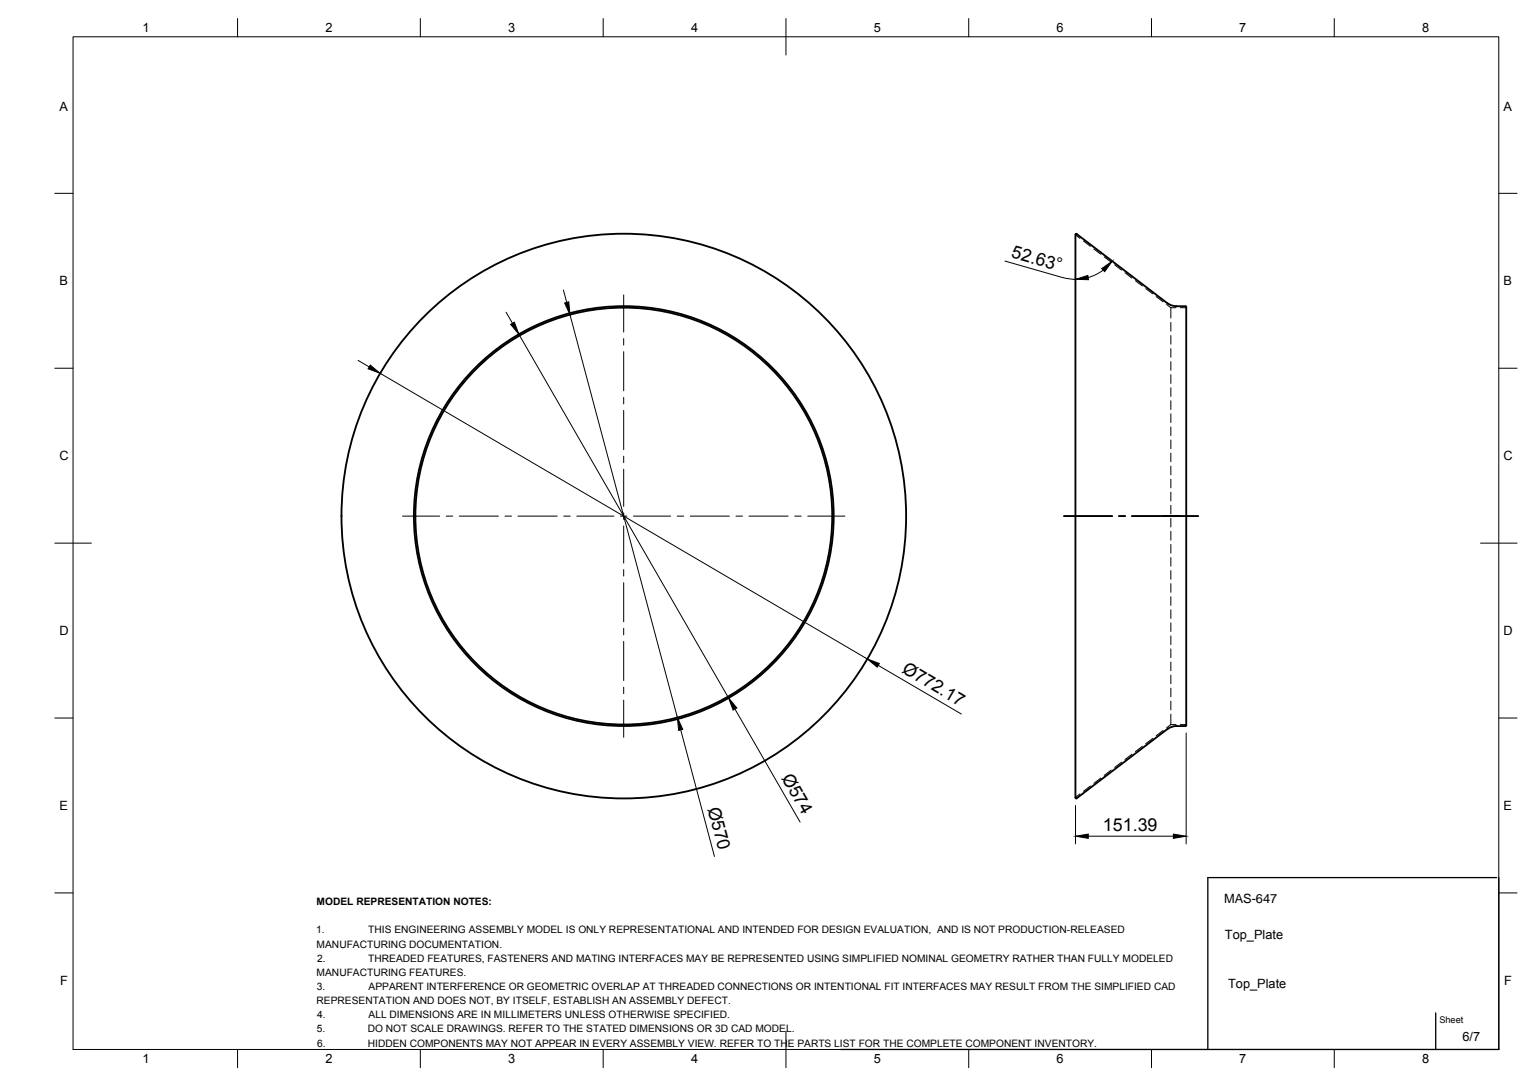
ISO-10303-21;
HEADER;
FILE_DESCRIPTION((''),'2;1');
FILE_NAME('Top_Plate.step','2026-10-09T11:36:02-07:00',(''),(''),'','','');
FILE_SCHEMA (('AUTOMOTIVE_DESIGN { 1 0 10303 214 3 1 1 }'));
ENDSEC;
DATA;
#10=MECHANICAL_DESIGN_GEOMETRIC_PRESENTATION_REPRESENTATION('',(#84),#1549);
#67=CONICAL_SURFACE('',#965,384.29203539823,0.652265221120532) ;
#68=CONICAL_SURFACE('',#974,287.,0.652265221120532) ;
#69=TOROIDAL_SURFACE('',#961,307.,20.) ;
#70=TOROIDAL_SURFACE('',#970,286.,1.) ;
#71=TOROIDAL_SURFACE('',#976,385.086746274481,0.99999999999999) ;
#74=SHAPE_REPRESENTATION_RELATIONSHIP('SRR','None',#1583,#79) ;
#79=ADVANCED_BREP_SHAPE_REPRESENTATION('',(#89),#1546) ;
#84=STYLED_ITEM('',(#1615),#89) ;
#89=MANIFOLD_SOLID_BREP('Body1',#846) ;
#161=FACE_OUTER_BOUND('',#235,.T.) ;
#162=FACE_OUTER_BOUND('',#236,.T.) ;
#163=FACE_OUTER_BOUND('',#237,.T.) ;
#164=FACE_OUTER_BOUND('',#238,.T.) ;
#165=FACE_OUTER_BOUND('',#239,.T.) ;
#166=FACE_OUTER_BOUND('',#240,.T.) ;
#167=FACE_OUTER_BOUND('',#241,.T.) ;
#235=EDGE_LOOP('',(#671,#672,#673,#674)) ;
#236=EDGE_LOOP('',(#675,#676,#677,#678)) ;
#237=EDGE_LOOP('',(#679,#680,#681,#682)) ;
#238=EDGE_LOOP('',(#683,#684,#685,#686)) ;
#239=EDGE_LOOP('',(#687,#688,#689,#690)) ;
#240=EDGE_LOOP('',(#691,#692,#693,#694)) ;
#241=EDGE_LOOP('',(#695,#696,#697,#698)) ;
#280=LINE('',#1421,#328) ;
#281=LINE('',#1426,#329) ;
#282=LINE('',#1432,#330) ;
#283=LINE('',#1436,#331) ;
#328=VECTOR('',#1163,384.29203539823) ;
#329=VECTOR('',#1170,285.) ;
#330=VECTOR('',#1179,287.) ;
#331=VECTOR('',#1184,287.) ;
#392=CIRCLE('',#962,291.105782474981) ;
#393=CIRCLE('',#963,20.) ;
#394=CIRCLE('',#964,287.) ;
#395=CIRCLE('',#966,285.) ;
#396=CIRCLE('',#967,384.29203539823) ;
#397=CIRCLE('',#969,285.) ;
#398=CIRCLE('',#971,287.) ;
#399=CIRCLE('',#972,1.) ;
#400=CIRCLE('',#975,385.881457150732) ;
#401=CIRCLE('',#977,0.99999999999999) ;
#444=VERTEX_POINT('',#1412) ;
#445=VERTEX_POINT('',#1414) ;
#446=VERTEX_POINT('',#1418) ;
#447=VERTEX_POINT('',#1420) ;
#448=VERTEX_POINT('',#1424) ;
#449=VERTEX_POINT('',#1428) ;
#450=VERTEX_POINT('',#1434) ;
#523=EDGE_CURVE('',#444,#444,#392,.T.) ;
#524=EDGE_CURVE('',#444,#445,#393,.T.) ;
#525=EDGE_CURVE('',#445,#445,#394,.T.) ;
#526=EDGE_CURVE('',#446,#446,#395,.T.) ;
#527=EDGE_CURVE('',#446,#447,#280,.T.) ;
#528=EDGE_CURVE('',#447,#447,#396,.T.) ;
#529=EDGE_CURVE('',#448,#448,#397,.T.) ;
#530=EDGE_CURVE('',#448,#446,#281,.T.) ;
#531=EDGE_CURVE('',#449,#449,#398,.T.) ;
#532=EDGE_CURVE('',#449,#448,#399,.T.) ;
#533=EDGE_CURVE('',#445,#449,#282,.T.) ;
#534=EDGE_CURVE('',#450,#450,#400,.T.) ;
#535=EDGE_CURVE('',#450,#444,#283,.T.) ;
#536=EDGE_CURVE('',#447,#450,#401,.T.) ;
#671=ORIENTED_EDGE('',*,*,#523,.F.) ;
#672=ORIENTED_EDGE('',*,*,#524,.T.) ;
#673=ORIENTED_EDGE('',*,*,#525,.F.) ;
#674=ORIENTED_EDGE('',*,*,#524,.F.) ;
#675=ORIENTED_EDGE('',*,*,#526,.F.) ;
#676=ORIENTED_EDGE('',*,*,#527,.T.) ;
#677=ORIENTED_EDGE('',*,*,#528,.T.) ;
#678=ORIENTED_EDGE('',*,*,#527,.F.) ;
#679=ORIENTED_EDGE('',*,*,#529,.F.) ;
#680=ORIENTED_EDGE('',*,*,#530,.T.) ;
#681=ORIENTED_EDGE('',*,*,#526,.T.) ;
#682=ORIENTED_EDGE('',*,*,#530,.F.) ;
#683=ORIENTED_EDGE('',*,*,#531,.F.) ;
#684=ORIENTED_EDGE('',*,*,#532,.T.) ;
#685=ORIENTED_EDGE('',*,*,#529,.T.) ;
#686=ORIENTED_EDGE('',*,*,#532,.F.) ;
#687=ORIENTED_EDGE('',*,*,#525,.T.) ;
#688=ORIENTED_EDGE('',*,*,#533,.T.) ;
#689=ORIENTED_EDGE('',*,*,#531,.T.) ;
#690=ORIENTED_EDGE('',*,*,#533,.F.) ;
#691=ORIENTED_EDGE('',*,*,#534,.F.) ;
#692=ORIENTED_EDGE('',*,*,#535,.T.) ;
#693=ORIENTED_EDGE('',*,*,#523,.T.) ;
#694=ORIENTED_EDGE('',*,*,#535,.F.) ;
#695=ORIENTED_EDGE('',*,*,#528,.F.) ;
#696=ORIENTED_EDGE('',*,*,#536,.T.) ;
#697=ORIENTED_EDGE('',*,*,#534,.T.) ;
#698=ORIENTED_EDGE('',*,*,#536,.F.) ;
#791=CYLINDRICAL_SURFACE('',#968,285.) ;
#792=CYLINDRICAL_SURFACE('',#973,287.) ;
#818=ADVANCED_FACE('',(#161),#69,.F.) ;
#819=ADVANCED_FACE('',(#162),#67,.F.) ;
#820=ADVANCED_FACE('',(#163),#791,.F.) ;
#821=ADVANCED_FACE('',(#164),#70,.T.) ;
#822=ADVANCED_FACE('',(#165),#792,.T.) ;
#823=ADVANCED_FACE('',(#166),#68,.T.) ;
#824=ADVANCED_FACE('',(#167),#71,.T.) ;
#846=CLOSED_SHELL('',(#818,#819,#820,#821,#822,#823,#824)) ;
#960=AXIS2_PLACEMENT_3D('',#1410,#1149,#1150) ;
#961=AXIS2_PLACEMENT_3D('',#1411,#1151,#1152) ;
#962=AXIS2_PLACEMENT_3D('',#1413,#1153,#1154) ;
#963=AXIS2_PLACEMENT_3D('',#1415,#1155,#1156) ;
#964=AXIS2_PLACEMENT_3D('',#1416,#1157,#1158) ;
#965=AXIS2_PLACEMENT_3D('',#1417,#1159,#1160) ;
#966=AXIS2_PLACEMENT_3D('',#1419,#1161,#1162) ;
#967=AXIS2_PLACEMENT_3D('',#1422,#1164,#1165) ;
#968=AXIS2_PLACEMENT_3D('',#1423,#1166,#1167) ;
#969=AXIS2_PLACEMENT_3D('',#1425,#1168,#1169) ;
#970=AXIS2_PLACEMENT_3D('',#1427,#1171,#1172) ;
#971=AXIS2_PLACEMENT_3D('',#1429,#1173,#1174) ;
#972=AXIS2_PLACEMENT_3D('',#1430,#1175,#1176) ;
#973=AXIS2_PLACEMENT_3D('',#1431,#1177,#1178) ;
#974=AXIS2_PLACEMENT_3D('',#1433,#1180,#1181) ;
#975=AXIS2_PLACEMENT_3D('',#1435,#1182,#1183) ;
#976=AXIS2_PLACEMENT_3D('',#1437,#1185,#1186) ;
#977=AXIS2_PLACEMENT_3D('',#1438,#1187,#1188) ;
#1149=DIRECTION('axis',(0.,0.,1.)) ;
#1150=DIRECTION('refdir',(1.,0.,0.)) ;
#1151=DIRECTION('center_axis',(0.,-1.,0.)) ;
#1152=DIRECTION('ref_axis',(0.,0.,-1.)) ;
#1153=DIRECTION('center_axis',(0.,-1.,0.)) ;
#1154=DIRECTION('ref_axis',(0.,0.,-1.)) ;
#1155=DIRECTION('center_axis',(1.,0.,1.22464679914735E-16)) ;
#1156=DIRECTION('ref_axis',(-1.22464679914735E-16,0.,1.)) ;
#1157=DIRECTION('center_axis',(0.,1.,0.)) ;
#1158=DIRECTION('ref_axis',(0.,0.,-1.)) ;
#1159=DIRECTION('center_axis',(0.,-1.,0.)) ;
#1160=DIRECTION('ref_axis',(0.,0.,-1.)) ;
#1161=DIRECTION('center_axis',(0.,-1.,0.)) ;
#1162=DIRECTION('ref_axis',(0.,0.,-1.)) ;
#1163=DIRECTION('',(-7.43346104024374E-17,-0.794710876250949,0.606988157354366)) ;
#1164=DIRECTION('center_axis',(0.,-1.,0.)) ;
#1165=DIRECTION('ref_axis',(0.,0.,-1.)) ;
#1166=DIRECTION('center_axis',(0.,-1.,0.)) ;
#1167=DIRECTION('ref_axis',(0.,0.,-1.)) ;
#1168=DIRECTION('center_axis',(0.,-1.,0.)) ;
#1169=DIRECTION('ref_axis',(0.,0.,-1.)) ;
#1170=DIRECTION('',(0.,-1.,0.)) ;
#1171=DIRECTION('center_axis',(0.,-1.,0.)) ;
#1172=DIRECTION('ref_axis',(0.,0.,-1.)) ;
#1173=DIRECTION('center_axis',(0.,-1.,0.)) ;
#1174=DIRECTION('ref_axis',(0.,0.,-1.)) ;
#1175=DIRECTION('center_axis',(-1.,0.,-1.22464679914735E-16)) ;
#1176=DIRECTION('ref_axis',(-1.22464679914735E-16,0.,1.)) ;
#1177=DIRECTION('center_axis',(0.,-1.,0.)) ;
#1178=DIRECTION('ref_axis',(0.,0.,-1.)) ;
#1179=DIRECTION('',(0.,1.,0.)) ;
#1180=DIRECTION('center_axis',(0.,-1.,0.)) ;
#1181=DIRECTION('ref_axis',(0.,0.,-1.)) ;
#1182=DIRECTION('center_axis',(0.,-1.,0.)) ;
#1183=DIRECTION('ref_axis',(0.,0.,-1.)) ;
#1184=DIRECTION('',(7.43346104024374E-17,0.794710876250949,-0.606988157354366)) ;
#1185=DIRECTION('center_axis',(0.,-1.,0.)) ;
#1186=DIRECTION('ref_axis',(0.,0.,-1.)) ;
#1187=DIRECTION('center_axis',(-1.,0.,-1.22464679914735E-16)) ;
#1188=DIRECTION('ref_axis',(-1.22464679914735E-16,0.,1.)) ;
#1410=CARTESIAN_POINT('',(0.,0.,0.)) ;
#1411=CARTESIAN_POINT('Origin',(0.,137.440607642436,0.)) ;
#1412=CARTESIAN_POINT('',(-3.56501764721271E-14,125.300844495349,291.105782474981)) ;
#1413=CARTESIAN_POINT('Origin',(0.,125.300844495349,0.)) ;
#1414=CARTESIAN_POINT('',(-3.5147363135529E-14,137.440607642436,287.)) ;
#1415=CARTESIAN_POINT('Origin',(-3.75966567338238E-14,137.440607642436,
307.)) ;
#1416=CARTESIAN_POINT('Origin',(0.,137.440607642436,0.)) ;
#1417=CARTESIAN_POINT('Origin',(0.,0.,0.)) ;
#1418=CARTESIAN_POINT('',(-3.49024337756996E-14,130.,285.)) ;
#1419=CARTESIAN_POINT('Origin',(0.,130.,0.)) ;
#1420=CARTESIAN_POINT('',(-4.70622011088264E-14,-3.6985068184911E-14,384.29203539823)) ;
#1421=CARTESIAN_POINT('',(-4.70622011088264E-14,0.,384.29203539823)) ;
#1422=CARTESIAN_POINT('Origin',(0.,0.,0.)) ;
#1423=CARTESIAN_POINT('Origin',(0.,0.,0.)) ;
#1424=CARTESIAN_POINT('',(-3.49024337756996E-14,150.,285.)) ;
#1425=CARTESIAN_POINT('Origin',(0.,150.,0.)) ;
#1426=CARTESIAN_POINT('',(-3.49024337756996E-14,0.,285.)) ;
#1427=CARTESIAN_POINT('Origin',(0.,150.,0.)) ;
#1428=CARTESIAN_POINT('',(-3.5147363135529E-14,150.,287.)) ;
#1429=CARTESIAN_POINT('Origin',(0.,150.,0.)) ;
#1430=CARTESIAN_POINT('Origin',(-3.50248984556143E-14,150.,286.)) ;
#1431=CARTESIAN_POINT('Origin',(0.,0.,0.)) ;
#1432=CARTESIAN_POINT('',(-3.5147363135529E-14,0.,287.)) ;
#1433=CARTESIAN_POINT('Origin',(0.,130.676418876585,0.)) ;
#1434=CARTESIAN_POINT('',(-4.7256849134996E-14,1.21397631470872,385.881457150732)) ;
#1435=CARTESIAN_POINT('Origin',(0.,1.21397631470873,0.)) ;
#1436=CARTESIAN_POINT('',(-3.5147363135529E-14,130.676418876585,287.)) ;
#1437=CARTESIAN_POINT('Origin',(0.,0.606988157354366,0.)) ;
#1438=CARTESIAN_POINT('Origin',(-4.71595251219112E-14,0.606988157354366,
385.086746274481)) ;
#1539=UNCERTAINTY_MEASURE_WITH_UNIT(LENGTH_MEASURE(0.01),#1550,
'DISTANCE_ACCURACY_VALUE',
'Maximum model space distance between geometric entities at asserted c
onnectivities') ;
#1542=UNCERTAINTY_MEASURE_WITH_UNIT(LENGTH_MEASURE(0.01),#1550,
'DISTANCE_ACCURACY_VALUE',
'Maximum model space distance between geometric entities at asserted c
onnectivities') ;
#1546=(
GEOMETRIC_REPRESENTATION_CONTEXT(3)
GLOBAL_UNCERTAINTY_ASSIGNED_CONTEXT((#1539))
GLOBAL_UNIT_ASSIGNED_CONTEXT((#1550,#1552,#1553))
REPRESENTATION_CONTEXT('','3D')
) ;
#1549=(
GEOMETRIC_REPRESENTATION_CONTEXT(3)
GLOBAL_UNCERTAINTY_ASSIGNED_CONTEXT((#1542))
GLOBAL_UNIT_ASSIGNED_CONTEXT((#1550,#1552,#1553))
REPRESENTATION_CONTEXT('','3D')
) ;
#1550=(
LENGTH_UNIT()
NAMED_UNIT(*)
SI_UNIT(.MILLI.,.METRE.)
) ;
#1552=(
NAMED_UNIT(*)
PLANE_ANGLE_UNIT()
SI_UNIT($,.RADIAN.)
) ;
#1553=(
NAMED_UNIT(*)
SI_UNIT($,.STERADIAN.)
SOLID_ANGLE_UNIT()
) ;
#1557=SHAPE_DEFINITION_REPRESENTATION(#1563,#1583) ;
#1563=PRODUCT_DEFINITION_SHAPE('',$,#1590) ;
#1583=SHAPE_REPRESENTATION('',(#960),#1546) ;
#1586=PRODUCT_DEFINITION_CONTEXT('part definition',#1606,'design') ;
#1590=PRODUCT_DEFINITION('Top_Plate','Top_Plate',#1596,#1586) ;
#1596=PRODUCT_DEFINITION_FORMATION('',$,#1611) ;
#1606=APPLICATION_CONTEXT(
'Core Data for Automotive Mechanical Design Process') ;
#1607=PRODUCT_CONTEXT('part definition',#1606,'mechanical') ;
#1611=PRODUCT('Top_Plate','Top_Plate',$,(#1607)) ;
#1615=PRESENTATION_STYLE_ASSIGNMENT((#1617)) ;
#1617=SURFACE_STYLE_USAGE(.BOTH.,#1619) ;
#1619=SURFACE_SIDE_STYLE('',(#1621)) ;
#1621=SURFACE_STYLE_FILL_AREA(#1623) ;
#1623=FILL_AREA_STYLE('Opaque(202,209,238)',(#1625)) ;
#1625=FILL_AREA_STYLE_COLOUR('Opaque(202,209,238)',#1627) ;
#1627=COLOUR_RGB('Opaque(202,209,238)', 0.09019608, 0.27058824, 0.51372549) ;
ENDSEC;
END-ISO-10303-21;
